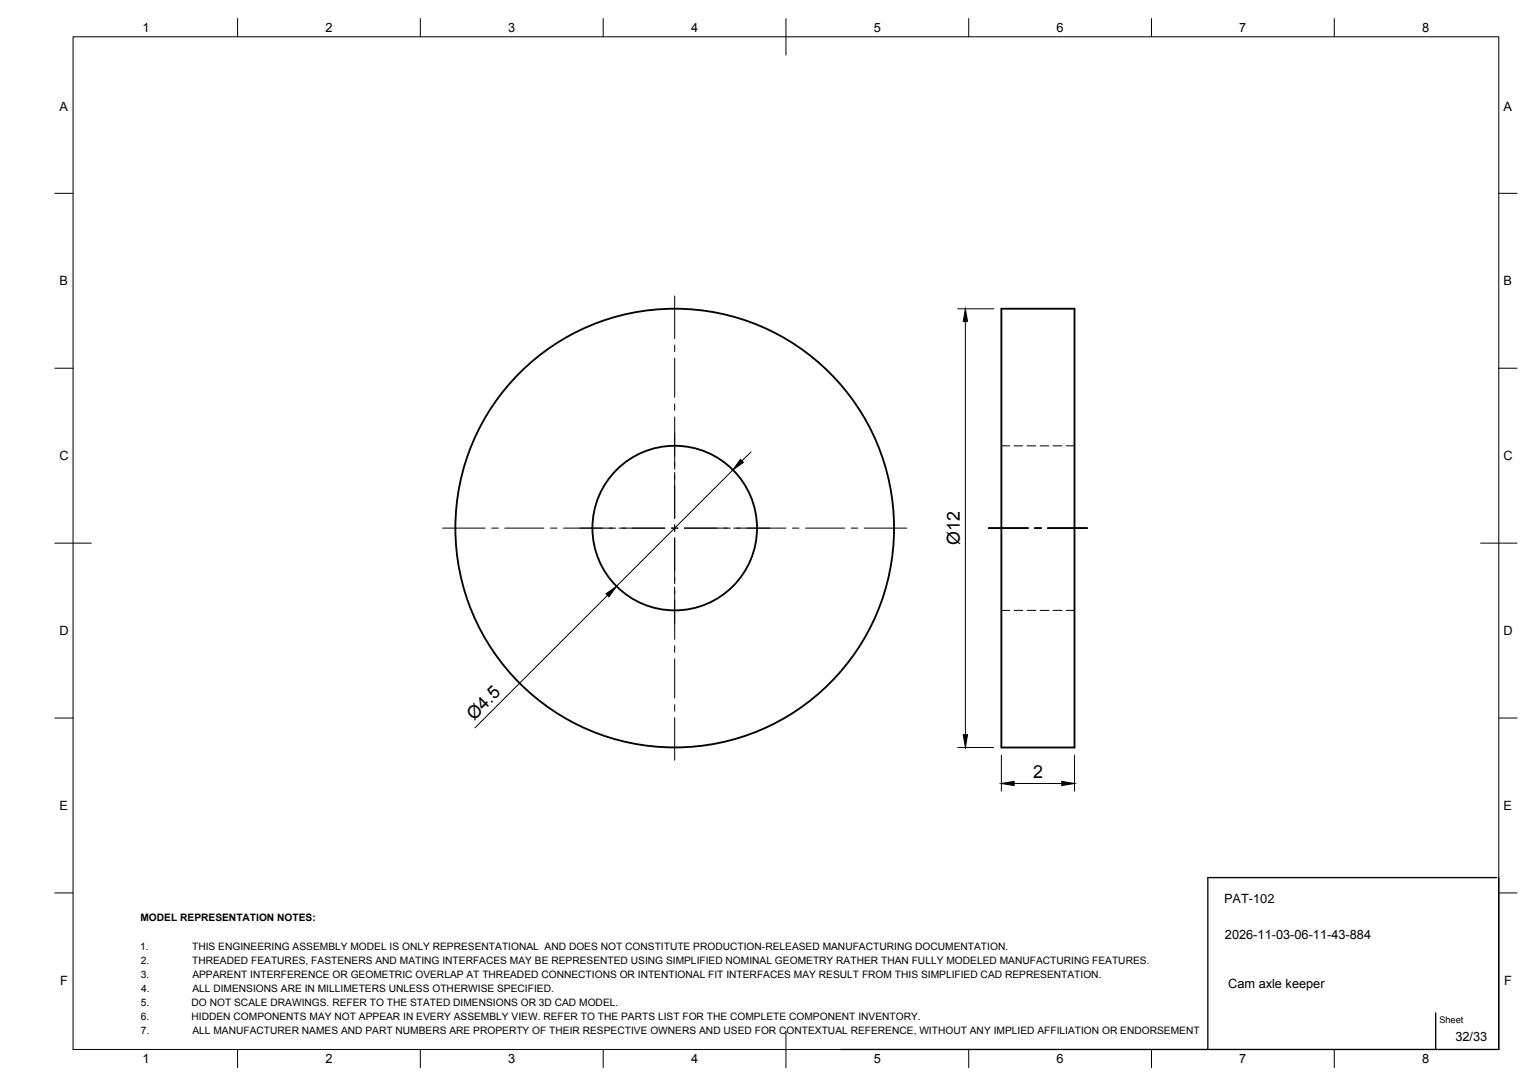
ISO-10303-21;
HEADER;
/* Generated by software containing ST-Developer
 * from STEP Tools, Inc. (www.steptools.com) 
 */

FILE_DESCRIPTION(
/* description */ ('Swing-away clamp arm'),
/* implementation_level */ '2;1');

FILE_NAME(
/* name */ 'Cam axle keeper.step',
/* time_stamp */ '2026-10-28T03:26:03-07:00',
/* author */ (''),
/* organization */ (''),
/* preprocessor_version */ 'ST-DEVELOPER v20.2',
/* originating_system */ 'Autodesk Translation Framework v15.17.0.0',
/* authorisation */ '');

FILE_SCHEMA (('AUTOMOTIVE_DESIGN { 1 0 10303 214 3 1 1 }'));
ENDSEC;

DATA;
#10=MECHANICAL_DESIGN_GEOMETRIC_PRESENTATION_REPRESENTATION('',(#323),#10627);
#263=SHAPE_REPRESENTATION_RELATIONSHIP('SRR','None',#10764,#289);
#289=ADVANCED_BREP_SHAPE_REPRESENTATION('',(#356),#10623);
#323=STYLED_ITEM('',(#10965),#356);
#356=MANIFOLD_SOLID_BREP('Body1',#4930);
#452=FACE_BOUND('',#1307,.T.);
#453=FACE_BOUND('',#1309,.T.);
#611=PLANE('',#5781);
#612=PLANE('',#5782);
#903=FACE_OUTER_BOUND('',#1304,.T.);
#904=FACE_OUTER_BOUND('',#1305,.T.);
#905=FACE_OUTER_BOUND('',#1306,.T.);
#906=FACE_OUTER_BOUND('',#1308,.T.);
#1304=EDGE_LOOP('',(#4349,#4350,#4351,#4352));
#1305=EDGE_LOOP('',(#4353,#4354,#4355,#4356));
#1306=EDGE_LOOP('',(#4357));
#1307=EDGE_LOOP('',(#4358));
#1308=EDGE_LOOP('',(#4359));
#1309=EDGE_LOOP('',(#4360));
#1622=LINE('',#10375,#1944);
#1623=LINE('',#10381,#1945);
#1944=VECTOR('',#7249,0.225);
#1945=VECTOR('',#7256,0.6);
#2239=CIRCLE('',#5776,0.225);
#2240=CIRCLE('',#5777,0.225);
#2241=CIRCLE('',#5779,0.6);
#2242=CIRCLE('',#5780,0.6);
#2626=VERTEX_POINT('',#10372);
#2627=VERTEX_POINT('',#10374);
#2628=VERTEX_POINT('',#10378);
#2629=VERTEX_POINT('',#10380);
#3207=EDGE_CURVE('',#2626,#2626,#2239,.T.);
#3208=EDGE_CURVE('',#2626,#2627,#1622,.T.);
#3209=EDGE_CURVE('',#2627,#2627,#2240,.T.);
#3210=EDGE_CURVE('',#2628,#2628,#2241,.T.);
#3211=EDGE_CURVE('',#2628,#2629,#1623,.T.);
#3212=EDGE_CURVE('',#2629,#2629,#2242,.T.);
#4349=ORIENTED_EDGE('',*,*,#3207,.F.);
#4350=ORIENTED_EDGE('',*,*,#3208,.T.);
#4351=ORIENTED_EDGE('',*,*,#3209,.T.);
#4352=ORIENTED_EDGE('',*,*,#3208,.F.);
#4353=ORIENTED_EDGE('',*,*,#3210,.F.);
#4354=ORIENTED_EDGE('',*,*,#3211,.T.);
#4355=ORIENTED_EDGE('',*,*,#3212,.T.);
#4356=ORIENTED_EDGE('',*,*,#3211,.F.);
#4357=ORIENTED_EDGE('',*,*,#3210,.T.);
#4358=ORIENTED_EDGE('',*,*,#3207,.T.);
#4359=ORIENTED_EDGE('',*,*,#3212,.F.);
#4360=ORIENTED_EDGE('',*,*,#3209,.F.);
#4584=CYLINDRICAL_SURFACE('',#5775,0.225);
#4585=CYLINDRICAL_SURFACE('',#5778,0.6);
#4858=ADVANCED_FACE('',(#903),#4584,.F.);
#4859=ADVANCED_FACE('',(#904),#4585,.T.);
#4860=ADVANCED_FACE('',(#905,#452),#611,.T.);
#4861=ADVANCED_FACE('',(#906,#453),#612,.F.);
#4930=CLOSED_SHELL('',(#4858,#4859,#4860,#4861));
#5774=AXIS2_PLACEMENT_3D('',#10370,#7243,#7244);
#5775=AXIS2_PLACEMENT_3D('',#10371,#7245,#7246);
#5776=AXIS2_PLACEMENT_3D('',#10373,#7247,#7248);
#5777=AXIS2_PLACEMENT_3D('',#10376,#7250,#7251);
#5778=AXIS2_PLACEMENT_3D('',#10377,#7252,#7253);
#5779=AXIS2_PLACEMENT_3D('',#10379,#7254,#7255);
#5780=AXIS2_PLACEMENT_3D('',#10382,#7257,#7258);
#5781=AXIS2_PLACEMENT_3D('',#10383,#7259,#7260);
#5782=AXIS2_PLACEMENT_3D('',#10384,#7261,#7262);
#7243=DIRECTION('axis',(0.,0.,1.));
#7244=DIRECTION('refdir',(1.,0.,0.));
#7245=DIRECTION('center_axis',(0.,1.,0.));
#7246=DIRECTION('ref_axis',(1.,0.,0.));
#7247=DIRECTION('center_axis',(0.,-1.,0.));
#7248=DIRECTION('ref_axis',(1.,0.,0.));
#7249=DIRECTION('',(0.,-1.,0.));
#7250=DIRECTION('center_axis',(0.,-1.,0.));
#7251=DIRECTION('ref_axis',(1.,0.,0.));
#7252=DIRECTION('center_axis',(0.,1.,0.));
#7253=DIRECTION('ref_axis',(1.,0.,0.));
#7254=DIRECTION('center_axis',(0.,1.,0.));
#7255=DIRECTION('ref_axis',(1.,0.,0.));
#7256=DIRECTION('',(0.,-1.,0.));
#7257=DIRECTION('center_axis',(0.,1.,0.));
#7258=DIRECTION('ref_axis',(1.,0.,0.));
#7259=DIRECTION('center_axis',(0.,1.,0.));
#7260=DIRECTION('ref_axis',(1.,0.,0.));
#7261=DIRECTION('center_axis',(0.,1.,0.));
#7262=DIRECTION('ref_axis',(1.,0.,0.));
#10370=CARTESIAN_POINT('',(0.,0.,0.));
#10371=CARTESIAN_POINT('Origin',(2.,-2.4,10.5));
#10372=CARTESIAN_POINT('',(1.775,-2.2,10.5));
#10373=CARTESIAN_POINT('Origin',(2.,-2.2,10.5));
#10374=CARTESIAN_POINT('',(1.775,-2.4,10.5));
#10375=CARTESIAN_POINT('',(1.775,-2.4,10.5));
#10376=CARTESIAN_POINT('Origin',(2.,-2.4,10.5));
#10377=CARTESIAN_POINT('Origin',(2.,-2.4,10.5));
#10378=CARTESIAN_POINT('',(1.4,-2.2,10.5));
#10379=CARTESIAN_POINT('Origin',(2.,-2.2,10.5));
#10380=CARTESIAN_POINT('',(1.4,-2.4,10.5));
#10381=CARTESIAN_POINT('',(1.4,-2.4,10.5));
#10382=CARTESIAN_POINT('Origin',(2.,-2.4,10.5));
#10383=CARTESIAN_POINT('Origin',(2.,-2.2,10.5));
#10384=CARTESIAN_POINT('Origin',(2.,-2.4,10.5));
#10591=UNCERTAINTY_MEASURE_WITH_UNIT(LENGTH_MEASURE(0.001),#10628,
'DISTANCE_ACCURACY_VALUE',
'Maximum model space distance between geometric entities at asserted c
onnectivities');
#10595=UNCERTAINTY_MEASURE_WITH_UNIT(LENGTH_MEASURE(0.001),#10628,
'DISTANCE_ACCURACY_VALUE',
'Maximum model space distance between geometric entities at asserted c
onnectivities');
#10623=(
GEOMETRIC_REPRESENTATION_CONTEXT(3)
GLOBAL_UNCERTAINTY_ASSIGNED_CONTEXT((#10591))
GLOBAL_UNIT_ASSIGNED_CONTEXT((#10628,#10630,#10631))
REPRESENTATION_CONTEXT('','3D')
);
#10627=(
GEOMETRIC_REPRESENTATION_CONTEXT(3)
GLOBAL_UNCERTAINTY_ASSIGNED_CONTEXT((#10595))
GLOBAL_UNIT_ASSIGNED_CONTEXT((#10628,#10630,#10631))
REPRESENTATION_CONTEXT('','3D')
);
#10628=(
LENGTH_UNIT()
NAMED_UNIT(*)
SI_UNIT(.CENTI.,.METRE.)
);
#10630=(
NAMED_UNIT(*)
PLANE_ANGLE_UNIT()
SI_UNIT($,.RADIAN.)
);
#10631=(
NAMED_UNIT(*)
SI_UNIT($,.STERADIAN.)
SOLID_ANGLE_UNIT()
);
#10659=SHAPE_DEFINITION_REPRESENTATION(#10705,#10764);
#10705=PRODUCT_DEFINITION_SHAPE('',$,#10796);
#10764=SHAPE_REPRESENTATION('',(#5774),#10623);
#10768=PRODUCT_DEFINITION_CONTEXT('part definition',#10863,'design');
#10796=PRODUCT_DEFINITION('Cam axle keeper','Cam axle keeper',#10827,#10768);
#10827=PRODUCT_DEFINITION_FORMATION('',$,#10892);
#10863=APPLICATION_CONTEXT(
'Core Data for Automotive Mechanical Design Process');
#10864=PRODUCT_CONTEXT('part definition',#10863,'mechanical');
#10892=PRODUCT('Cam axle keeper','Cam axle keeper','Cam axle keeper',(#10864));
#10959=COLOUR_RGB('Grey',0.48,0.52,0.57);
#10960=FILL_AREA_STYLE_COLOUR('',#10959);
#10961=FILL_AREA_STYLE('',(#10960));
#10962=SURFACE_STYLE_FILL_AREA(#10961);
#10963=SURFACE_SIDE_STYLE('',(#10962));
#10964=SURFACE_STYLE_USAGE(.BOTH.,#10963);
#10965=PRESENTATION_STYLE_ASSIGNMENT((#10964));
ENDSEC;
END-ISO-10303-21;
